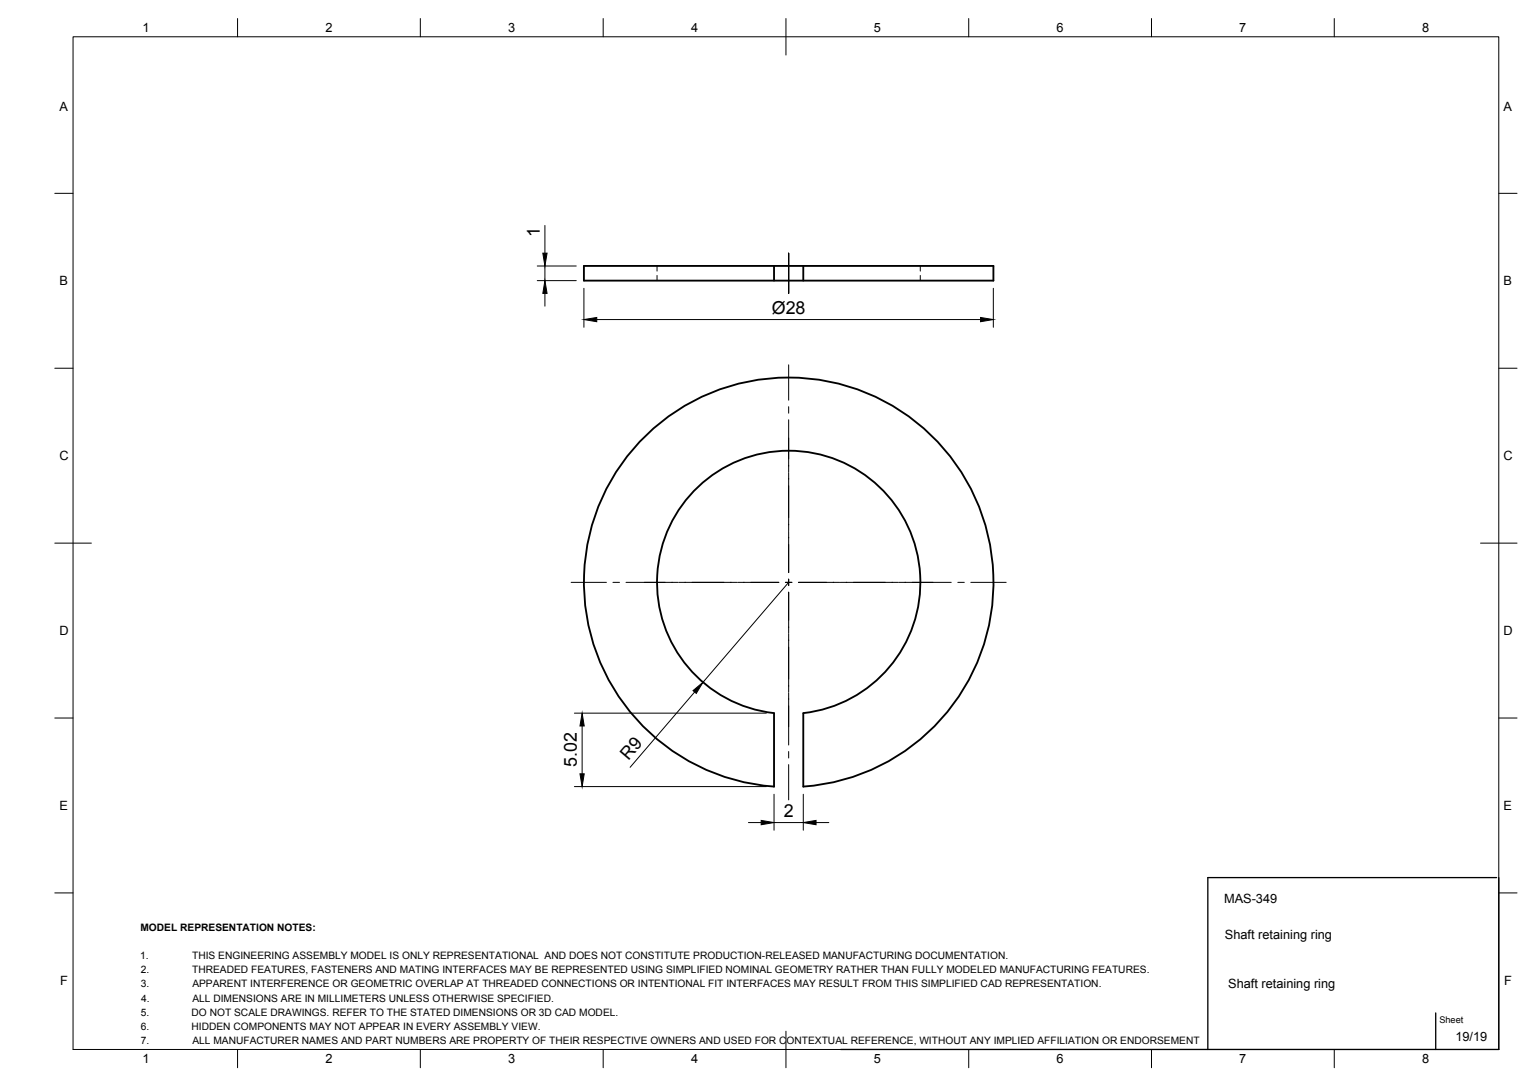
ISO-10303-21;
HEADER;
/* Generated by software containing ST-Developer
 * from STEP Tools, Inc. (www.steptools.com) 
 */

FILE_DESCRIPTION(
/* description */ ('Independent two-stage semi-open centrifugal-pump CAD. Shared impeller
s, open-machinable return casings, removable diaphragms, bronze wear/j
ournal rings, volume-preserving seal instances, retained keyed shaft, 
opposed mechanical face rings and partly threaded tie hardware. Native
 shaft rotation. Geometric topology/clearance only; flow/head/efficien
cy, pressure, cavitation, balance, preload, face loading and secondary
 seal fits/bonds, material/thermal/tolerance selection and life unassi
gned. External drive, coupling, anchors and piping bolts omitted.'),
/* implementation_level */ '2;1');

FILE_NAME(
/* name */ 'Shaft retaining ring.step',
/* time_stamp */ '2026-11-08T18:06:32-08:00',
/* author */ (''),
/* organization */ (''),
/* preprocessor_version */ 'ST-DEVELOPER v20.2',
/* originating_system */ 'Autodesk Translation Framework v15.17.0.0',
/* authorisation */ '');

FILE_SCHEMA (('AUTOMOTIVE_DESIGN { 1 0 10303 214 3 1 1 }'));
ENDSEC;

DATA;
#10=MECHANICAL_DESIGN_GEOMETRIC_PRESENTATION_REPRESENTATION('',(#410),#16687);
#372=SHAPE_REPRESENTATION_RELATIONSHIP('SRR','None',#16781,#391);
#391=ADVANCED_BREP_SHAPE_REPRESENTATION('',(#429),#16685);
#410=STYLED_ITEM('',(#16880),#429);
#429=MANIFOLD_SOLID_BREP('Body1',#6129);
#671=PLANE('',#6908);
#672=PLANE('',#6909);
#673=PLANE('',#6910);
#674=PLANE('',#6917);
#996=FACE_OUTER_BOUND('',#1463,.T.);
#997=FACE_OUTER_BOUND('',#1464,.T.);
#998=FACE_OUTER_BOUND('',#1465,.T.);
#999=FACE_OUTER_BOUND('',#1466,.T.);
#1000=FACE_OUTER_BOUND('',#1467,.T.);
#1001=FACE_OUTER_BOUND('',#1468,.T.);
#1463=EDGE_LOOP('',(#5377,#5378,#5379,#5380));
#1464=EDGE_LOOP('',(#5381,#5382,#5383,#5384));
#1465=EDGE_LOOP('',(#5385,#5386,#5387,#5388));
#1466=EDGE_LOOP('',(#5389,#5390,#5391,#5392));
#1467=EDGE_LOOP('',(#5393,#5394,#5395,#5396));
#1468=EDGE_LOOP('',(#5397,#5398,#5399,#5400));
#1828=LINE('',#15251,#2197);
#1829=LINE('',#15253,#2198);
#1830=LINE('',#15255,#2199);
#1831=LINE('',#15256,#2200);
#1832=LINE('',#15260,#2201);
#1833=LINE('',#15262,#2202);
#1834=LINE('',#15264,#2203);
#1835=LINE('',#15265,#2204);
#2197=VECTOR('',#8450,1.);
#2198=VECTOR('',#8451,1.);
#2199=VECTOR('',#8452,1.);
#2200=VECTOR('',#8453,1.);
#2201=VECTOR('',#8456,1.);
#2202=VECTOR('',#8457,1.);
#2203=VECTOR('',#8458,1.);
#2204=VECTOR('',#8459,1.);
#2486=CIRCLE('',#6911,1.4);
#2487=CIRCLE('',#6912,0.9);
#2488=CIRCLE('',#6914,0.9);
#2489=CIRCLE('',#6916,1.4);
#2993=VERTEX_POINT('',#15249);
#2994=VERTEX_POINT('',#15250);
#2995=VERTEX_POINT('',#15252);
#2996=VERTEX_POINT('',#15254);
#2997=VERTEX_POINT('',#15258);
#2998=VERTEX_POINT('',#15259);
#2999=VERTEX_POINT('',#15261);
#3000=VERTEX_POINT('',#15263);
#3798=EDGE_CURVE('',#2993,#2994,#1828,.T.);
#3799=EDGE_CURVE('',#2995,#2993,#1829,.T.);
#3800=EDGE_CURVE('',#2996,#2995,#1830,.T.);
#3801=EDGE_CURVE('',#2994,#2996,#1831,.T.);
#3802=EDGE_CURVE('',#2997,#2998,#1832,.T.);
#3803=EDGE_CURVE('',#2999,#2997,#1833,.T.);
#3804=EDGE_CURVE('',#3000,#2999,#1834,.T.);
#3805=EDGE_CURVE('',#2998,#3000,#1835,.T.);
#3806=EDGE_CURVE('',#2995,#3000,#2486,.T.);
#3807=EDGE_CURVE('',#2998,#2993,#2487,.T.);
#3808=EDGE_CURVE('',#2997,#2994,#2488,.T.);
#3809=EDGE_CURVE('',#2996,#2999,#2489,.T.);
#5377=ORIENTED_EDGE('',*,*,#3798,.F.);
#5378=ORIENTED_EDGE('',*,*,#3799,.F.);
#5379=ORIENTED_EDGE('',*,*,#3800,.F.);
#5380=ORIENTED_EDGE('',*,*,#3801,.F.);
#5381=ORIENTED_EDGE('',*,*,#3802,.F.);
#5382=ORIENTED_EDGE('',*,*,#3803,.F.);
#5383=ORIENTED_EDGE('',*,*,#3804,.F.);
#5384=ORIENTED_EDGE('',*,*,#3805,.F.);
#5385=ORIENTED_EDGE('',*,*,#3805,.T.);
#5386=ORIENTED_EDGE('',*,*,#3806,.F.);
#5387=ORIENTED_EDGE('',*,*,#3799,.T.);
#5388=ORIENTED_EDGE('',*,*,#3807,.F.);
#5389=ORIENTED_EDGE('',*,*,#3802,.T.);
#5390=ORIENTED_EDGE('',*,*,#3807,.T.);
#5391=ORIENTED_EDGE('',*,*,#3798,.T.);
#5392=ORIENTED_EDGE('',*,*,#3808,.F.);
#5393=ORIENTED_EDGE('',*,*,#3804,.T.);
#5394=ORIENTED_EDGE('',*,*,#3809,.F.);
#5395=ORIENTED_EDGE('',*,*,#3800,.T.);
#5396=ORIENTED_EDGE('',*,*,#3806,.T.);
#5397=ORIENTED_EDGE('',*,*,#3803,.T.);
#5398=ORIENTED_EDGE('',*,*,#3808,.T.);
#5399=ORIENTED_EDGE('',*,*,#3801,.T.);
#5400=ORIENTED_EDGE('',*,*,#3809,.T.);
#5746=CYLINDRICAL_SURFACE('',#6913,0.9);
#5747=CYLINDRICAL_SURFACE('',#6915,1.4);
#6075=ADVANCED_FACE('',(#996),#671,.F.);
#6076=ADVANCED_FACE('',(#997),#672,.F.);
#6077=ADVANCED_FACE('',(#998),#673,.F.);
#6078=ADVANCED_FACE('',(#999),#5746,.F.);
#6079=ADVANCED_FACE('',(#1000),#5747,.T.);
#6080=ADVANCED_FACE('',(#1001),#674,.T.);
#6129=CLOSED_SHELL('',(#6075,#6076,#6077,#6078,#6079,#6080));
#6907=AXIS2_PLACEMENT_3D('',#15247,#8446,#8447);
#6908=AXIS2_PLACEMENT_3D('',#15248,#8448,#8449);
#6909=AXIS2_PLACEMENT_3D('',#15257,#8454,#8455);
#6910=AXIS2_PLACEMENT_3D('',#15266,#8460,#8461);
#6911=AXIS2_PLACEMENT_3D('',#15267,#8462,#8463);
#6912=AXIS2_PLACEMENT_3D('',#15268,#8464,#8465);
#6913=AXIS2_PLACEMENT_3D('',#15269,#8466,#8467);
#6914=AXIS2_PLACEMENT_3D('',#15270,#8468,#8469);
#6915=AXIS2_PLACEMENT_3D('',#15271,#8470,#8471);
#6916=AXIS2_PLACEMENT_3D('',#15272,#8472,#8473);
#6917=AXIS2_PLACEMENT_3D('',#15273,#8474,#8475);
#8446=DIRECTION('axis',(0.,0.,1.));
#8447=DIRECTION('refdir',(1.,0.,0.));
#8448=DIRECTION('center_axis',(-1.,0.,0.));
#8449=DIRECTION('ref_axis',(0.,1.,0.));
#8450=DIRECTION('',(0.,0.,1.));
#8451=DIRECTION('',(0.,-1.,0.));
#8452=DIRECTION('',(0.,0.,-1.));
#8453=DIRECTION('',(0.,1.,0.));
#8454=DIRECTION('center_axis',(1.,0.,0.));
#8455=DIRECTION('ref_axis',(0.,-1.,0.));
#8456=DIRECTION('',(0.,0.,-1.));
#8457=DIRECTION('',(0.,-1.,0.));
#8458=DIRECTION('',(0.,0.,1.));
#8459=DIRECTION('',(0.,1.,0.));
#8460=DIRECTION('center_axis',(0.,0.,1.));
#8461=DIRECTION('ref_axis',(1.,0.,0.));
#8462=DIRECTION('center_axis',(0.,0.,1.));
#8463=DIRECTION('ref_axis',(1.,0.,0.));
#8464=DIRECTION('center_axis',(0.,0.,-1.));
#8465=DIRECTION('ref_axis',(1.,0.,0.));
#8466=DIRECTION('center_axis',(0.,0.,1.));
#8467=DIRECTION('ref_axis',(6.12323399573677E-17,-1.,0.));
#8468=DIRECTION('center_axis',(0.,0.,-1.));
#8469=DIRECTION('ref_axis',(1.,0.,0.));
#8470=DIRECTION('center_axis',(0.,0.,1.));
#8471=DIRECTION('ref_axis',(6.12323399573677E-17,-1.,0.));
#8472=DIRECTION('center_axis',(0.,0.,1.));
#8473=DIRECTION('ref_axis',(1.,0.,0.));
#8474=DIRECTION('center_axis',(0.,0.,1.));
#8475=DIRECTION('ref_axis',(1.,0.,0.));
#15247=CARTESIAN_POINT('',(0.,0.,0.));
#15248=CARTESIAN_POINT('Origin',(-0.1,0.,0.1));
#15249=CARTESIAN_POINT('',(-0.1,0.894427190999916,0.));
#15250=CARTESIAN_POINT('',(-0.1,0.894427190999916,0.1));
#15251=CARTESIAN_POINT('',(-0.1,0.894427190999916,0.));
#15252=CARTESIAN_POINT('',(-0.1,1.39642400437689,0.));
#15253=CARTESIAN_POINT('',(-0.1,0.,0.));
#15254=CARTESIAN_POINT('',(-0.1,1.39642400437689,0.1));
#15255=CARTESIAN_POINT('',(-0.1,1.39642400437689,0.));
#15256=CARTESIAN_POINT('',(-0.1,0.,0.1));
#15257=CARTESIAN_POINT('Origin',(0.1,2.8,0.1));
#15258=CARTESIAN_POINT('',(0.1,0.894427190999916,0.1));
#15259=CARTESIAN_POINT('',(0.1,0.894427190999916,0.));
#15260=CARTESIAN_POINT('',(0.1,0.894427190999916,0.));
#15261=CARTESIAN_POINT('',(0.1,1.39642400437689,0.1));
#15262=CARTESIAN_POINT('',(0.1,1.4,0.1));
#15263=CARTESIAN_POINT('',(0.1,1.39642400437689,0.));
#15264=CARTESIAN_POINT('',(0.1,1.39642400437689,0.));
#15265=CARTESIAN_POINT('',(0.1,1.4,0.));
#15266=CARTESIAN_POINT('Origin',(0.,0.,0.));
#15267=CARTESIAN_POINT('Origin',(0.,0.,0.));
#15268=CARTESIAN_POINT('Origin',(0.,0.,0.));
#15269=CARTESIAN_POINT('Origin',(0.,0.,0.));
#15270=CARTESIAN_POINT('Origin',(0.,0.,0.1));
#15271=CARTESIAN_POINT('Origin',(0.,0.,0.));
#15272=CARTESIAN_POINT('Origin',(0.,0.,0.1));
#15273=CARTESIAN_POINT('Origin',(0.,0.,0.1));
#16664=UNCERTAINTY_MEASURE_WITH_UNIT(LENGTH_MEASURE(0.001),#16688,
'DISTANCE_ACCURACY_VALUE',
'Maximum model space distance between geometric entities at asserted c
onnectivities');
#16666=UNCERTAINTY_MEASURE_WITH_UNIT(LENGTH_MEASURE(0.001),#16688,
'DISTANCE_ACCURACY_VALUE',
'Maximum model space distance between geometric entities at asserted c
onnectivities');
#16685=(
GEOMETRIC_REPRESENTATION_CONTEXT(3)
GLOBAL_UNCERTAINTY_ASSIGNED_CONTEXT((#16664))
GLOBAL_UNIT_ASSIGNED_CONTEXT((#16688,#16690,#16691))
REPRESENTATION_CONTEXT('','3D')
);
#16687=(
GEOMETRIC_REPRESENTATION_CONTEXT(3)
GLOBAL_UNCERTAINTY_ASSIGNED_CONTEXT((#16666))
GLOBAL_UNIT_ASSIGNED_CONTEXT((#16688,#16690,#16691))
REPRESENTATION_CONTEXT('','3D')
);
#16688=(
LENGTH_UNIT()
NAMED_UNIT(*)
SI_UNIT(.CENTI.,.METRE.)
);
#16690=(
NAMED_UNIT(*)
PLANE_ANGLE_UNIT()
SI_UNIT($,.RADIAN.)
);
#16691=(
NAMED_UNIT(*)
SI_UNIT($,.STERADIAN.)
SOLID_ANGLE_UNIT()
);
#16710=SHAPE_DEFINITION_REPRESENTATION(#16730,#16781);
#16730=PRODUCT_DEFINITION_SHAPE('',$,#16802);
#16781=SHAPE_REPRESENTATION('',(#6907),#16685);
#16783=PRODUCT_DEFINITION_CONTEXT('part definition',#16845,'design');
#16802=PRODUCT_DEFINITION('Shaft retaining ring','Shaft retaining ring',
#16822,#16783);
#16822=PRODUCT_DEFINITION_FORMATION('',$,#16865);
#16845=APPLICATION_CONTEXT(
'Core Data for Automotive Mechanical Design Process');
#16846=PRODUCT_CONTEXT('part definition',#16845,'mechanical');
#16865=PRODUCT('Shaft retaining ring','Shaft retaining ring',$,(#16846));
#16880=PRESENTATION_STYLE_ASSIGNMENT((#16895));
#16895=SURFACE_STYLE_USAGE(.BOTH.,#16910);
#16910=SURFACE_SIDE_STYLE('',(#16925));
#16925=SURFACE_STYLE_FILL_AREA(#16940);
#16940=FILL_AREA_STYLE('Dark gray',(#16955));
#16955=FILL_AREA_STYLE_COLOUR('Dark gray',#16970);
#16970=COLOUR_RGB('Dark gray',0.250980392156863,0.282352941176471,0.32156862745098);
ENDSEC;
END-ISO-10303-21;
